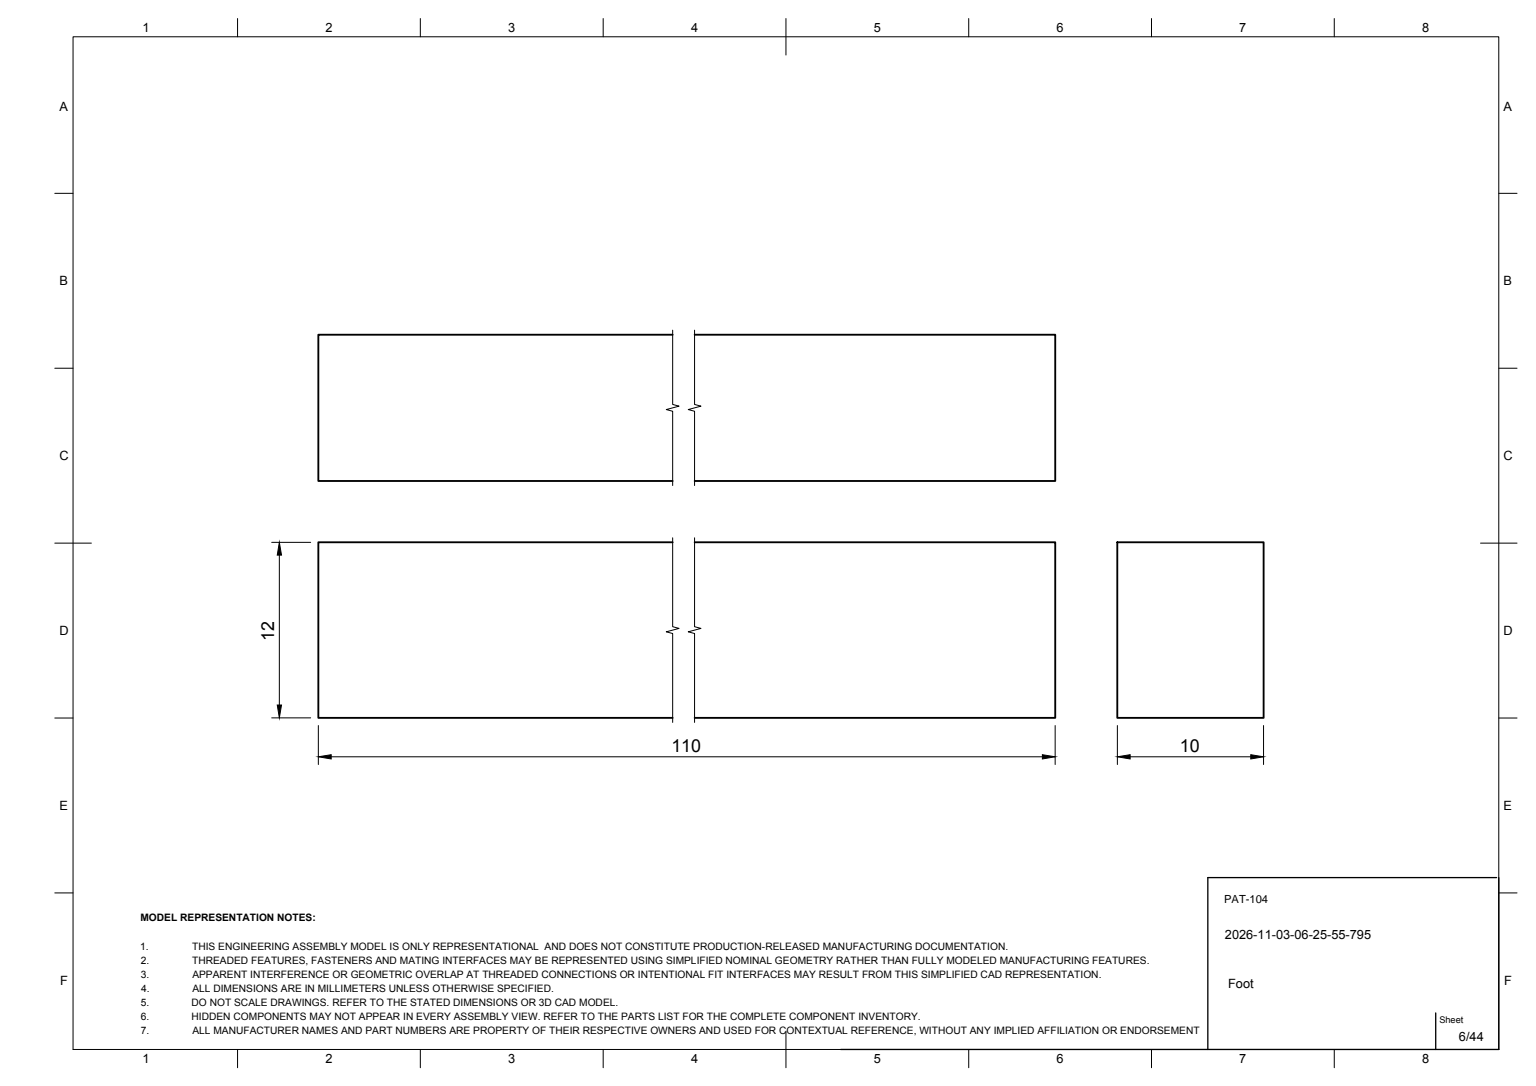
ISO-10303-21;
HEADER;
/* Generated by software containing ST-Developer
 * from STEP Tools, Inc. (www.steptools.com) 
 */

FILE_DESCRIPTION(
/* description */ ('Timing belt drive module 2 mm Pitch Timing 20T-40T'),

/* implementation_level */ '2;1');

FILE_NAME(
/* name */ 'Foot.step',
/* time_stamp */ '2026-10-28T03:25:12-07:00',
/* author */ (''),
/* organization */ (''),
/* preprocessor_version */ 'ST-DEVELOPER v20.2',
/* originating_system */ 'Autodesk Translation Framework v15.17.0.0',
/* authorisation */ '');

FILE_SCHEMA (('AUTOMOTIVE_DESIGN { 1 0 10303 214 3 1 1 }'));
ENDSEC;

DATA;
#10=MECHANICAL_DESIGN_GEOMETRIC_PRESENTATION_REPRESENTATION('',(#525),#17830);
#439=SHAPE_REPRESENTATION_RELATIONSHIP('SRR','None',#18009,#482);
#482=ADVANCED_BREP_SHAPE_REPRESENTATION('',(#583),#17784);
#525=STYLED_ITEM('',(#18331),#583);
#583=MANIFOLD_SOLID_BREP('Body1',#8982);
#791=PLANE('',#9578);
#792=PLANE('',#9579);
#793=PLANE('',#9580);
#794=PLANE('',#9581);
#795=PLANE('',#9582);
#796=PLANE('',#9583);
#992=FACE_OUTER_BOUND('',#1523,.T.);
#993=FACE_OUTER_BOUND('',#1524,.T.);
#994=FACE_OUTER_BOUND('',#1525,.T.);
#995=FACE_OUTER_BOUND('',#1526,.T.);
#996=FACE_OUTER_BOUND('',#1527,.T.);
#997=FACE_OUTER_BOUND('',#1528,.T.);
#1523=EDGE_LOOP('',(#5929,#5930,#5931,#5932));
#1524=EDGE_LOOP('',(#5933,#5934,#5935,#5936));
#1525=EDGE_LOOP('',(#5937,#5938,#5939,#5940));
#1526=EDGE_LOOP('',(#5941,#5942,#5943,#5944));
#1527=EDGE_LOOP('',(#5945,#5946,#5947,#5948));
#1528=EDGE_LOOP('',(#5949,#5950,#5951,#5952));
#2840=LINE('',#14040,#3318);
#2841=LINE('',#14042,#3319);
#2842=LINE('',#14044,#3320);
#2843=LINE('',#14045,#3321);
#2844=LINE('',#14048,#3322);
#2845=LINE('',#14050,#3323);
#2846=LINE('',#14051,#3324);
#2847=LINE('',#14054,#3325);
#2848=LINE('',#14056,#3326);
#2849=LINE('',#14057,#3327);
#2850=LINE('',#14059,#3328);
#2851=LINE('',#14060,#3329);
#3318=VECTOR('',#10985,1.);
#3319=VECTOR('',#10986,1.);
#3320=VECTOR('',#10987,1.);
#3321=VECTOR('',#10988,1.);
#3322=VECTOR('',#10991,1.);
#3323=VECTOR('',#10992,1.);
#3324=VECTOR('',#10993,1.);
#3325=VECTOR('',#10996,1.);
#3326=VECTOR('',#10997,1.);
#3327=VECTOR('',#10998,1.);
#3328=VECTOR('',#11001,1.);
#3329=VECTOR('',#11002,1.);
#3798=VERTEX_POINT('',#14038);
#3799=VERTEX_POINT('',#14039);
#3800=VERTEX_POINT('',#14041);
#3801=VERTEX_POINT('',#14043);
#3802=VERTEX_POINT('',#14047);
#3803=VERTEX_POINT('',#14049);
#3804=VERTEX_POINT('',#14053);
#3805=VERTEX_POINT('',#14055);
#4647=EDGE_CURVE('',#3798,#3799,#2840,.T.);
#4648=EDGE_CURVE('',#3799,#3800,#2841,.T.);
#4649=EDGE_CURVE('',#3801,#3800,#2842,.T.);
#4650=EDGE_CURVE('',#3798,#3801,#2843,.T.);
#4651=EDGE_CURVE('',#3802,#3798,#2844,.T.);
#4652=EDGE_CURVE('',#3803,#3801,#2845,.T.);
#4653=EDGE_CURVE('',#3802,#3803,#2846,.T.);
#4654=EDGE_CURVE('',#3804,#3802,#2847,.T.);
#4655=EDGE_CURVE('',#3805,#3803,#2848,.T.);
#4656=EDGE_CURVE('',#3804,#3805,#2849,.T.);
#4657=EDGE_CURVE('',#3799,#3804,#2850,.T.);
#4658=EDGE_CURVE('',#3800,#3805,#2851,.T.);
#5929=ORIENTED_EDGE('',*,*,#4647,.T.);
#5930=ORIENTED_EDGE('',*,*,#4648,.T.);
#5931=ORIENTED_EDGE('',*,*,#4649,.F.);
#5932=ORIENTED_EDGE('',*,*,#4650,.F.);
#5933=ORIENTED_EDGE('',*,*,#4651,.T.);
#5934=ORIENTED_EDGE('',*,*,#4650,.T.);
#5935=ORIENTED_EDGE('',*,*,#4652,.F.);
#5936=ORIENTED_EDGE('',*,*,#4653,.F.);
#5937=ORIENTED_EDGE('',*,*,#4654,.T.);
#5938=ORIENTED_EDGE('',*,*,#4653,.T.);
#5939=ORIENTED_EDGE('',*,*,#4655,.F.);
#5940=ORIENTED_EDGE('',*,*,#4656,.F.);
#5941=ORIENTED_EDGE('',*,*,#4657,.T.);
#5942=ORIENTED_EDGE('',*,*,#4656,.T.);
#5943=ORIENTED_EDGE('',*,*,#4658,.F.);
#5944=ORIENTED_EDGE('',*,*,#4648,.F.);
#5945=ORIENTED_EDGE('',*,*,#4658,.T.);
#5946=ORIENTED_EDGE('',*,*,#4655,.T.);
#5947=ORIENTED_EDGE('',*,*,#4652,.T.);
#5948=ORIENTED_EDGE('',*,*,#4649,.T.);
#5949=ORIENTED_EDGE('',*,*,#4657,.F.);
#5950=ORIENTED_EDGE('',*,*,#4647,.F.);
#5951=ORIENTED_EDGE('',*,*,#4651,.F.);
#5952=ORIENTED_EDGE('',*,*,#4654,.F.);
#8490=ADVANCED_FACE('',(#992),#791,.T.);
#8491=ADVANCED_FACE('',(#993),#792,.T.);
#8492=ADVANCED_FACE('',(#994),#793,.T.);
#8493=ADVANCED_FACE('',(#995),#794,.T.);
#8494=ADVANCED_FACE('',(#996),#795,.T.);
#8495=ADVANCED_FACE('',(#997),#796,.F.);
#8982=CLOSED_SHELL('',(#8490,#8491,#8492,#8493,#8494,#8495));
#9577=AXIS2_PLACEMENT_3D('',#14036,#10981,#10982);
#9578=AXIS2_PLACEMENT_3D('',#14037,#10983,#10984);
#9579=AXIS2_PLACEMENT_3D('',#14046,#10989,#10990);
#9580=AXIS2_PLACEMENT_3D('',#14052,#10994,#10995);
#9581=AXIS2_PLACEMENT_3D('',#14058,#10999,#11000);
#9582=AXIS2_PLACEMENT_3D('',#14061,#11003,#11004);
#9583=AXIS2_PLACEMENT_3D('',#14062,#11005,#11006);
#10981=DIRECTION('axis',(0.,0.,1.));
#10982=DIRECTION('refdir',(1.,0.,0.));
#10983=DIRECTION('center_axis',(0.,1.,0.));
#10984=DIRECTION('ref_axis',(-1.,0.,0.));
#10985=DIRECTION('',(-1.,0.,0.));
#10986=DIRECTION('',(0.,0.,1.));
#10987=DIRECTION('',(-1.,0.,0.));
#10988=DIRECTION('',(0.,0.,1.));
#10989=DIRECTION('center_axis',(1.,0.,0.));
#10990=DIRECTION('ref_axis',(0.,1.,0.));
#10991=DIRECTION('',(0.,1.,0.));
#10992=DIRECTION('',(0.,1.,0.));
#10993=DIRECTION('',(0.,0.,1.));
#10994=DIRECTION('center_axis',(0.,-1.,0.));
#10995=DIRECTION('ref_axis',(1.,0.,0.));
#10996=DIRECTION('',(1.,0.,0.));
#10997=DIRECTION('',(1.,0.,0.));
#10998=DIRECTION('',(0.,0.,1.));
#10999=DIRECTION('center_axis',(-1.,0.,0.));
#11000=DIRECTION('ref_axis',(0.,-1.,0.));
#11001=DIRECTION('',(0.,-1.,0.));
#11002=DIRECTION('',(0.,-1.,0.));
#11003=DIRECTION('center_axis',(0.,0.,1.));
#11004=DIRECTION('ref_axis',(1.,0.,0.));
#11005=DIRECTION('center_axis',(0.,0.,1.));
#11006=DIRECTION('ref_axis',(1.,0.,0.));
#14036=CARTESIAN_POINT('',(0.,0.,0.));
#14037=CARTESIAN_POINT('Origin',(-3.,4.5,-2.4));
#14038=CARTESIAN_POINT('',(-3.,4.5,-2.4));
#14039=CARTESIAN_POINT('',(-4.,4.5,-2.4));
#14040=CARTESIAN_POINT('',(-3.,4.5,-2.4));
#14041=CARTESIAN_POINT('',(-4.,4.5,-1.2));
#14042=CARTESIAN_POINT('',(-4.,4.5,-2.4));
#14043=CARTESIAN_POINT('',(-3.,4.5,-1.2));
#14044=CARTESIAN_POINT('',(-3.,4.5,-1.2));
#14045=CARTESIAN_POINT('',(-3.,4.5,-2.4));
#14046=CARTESIAN_POINT('Origin',(-3.,-6.5,-2.4));
#14047=CARTESIAN_POINT('',(-3.,-6.5,-2.4));
#14048=CARTESIAN_POINT('',(-3.,-6.5,-2.4));
#14049=CARTESIAN_POINT('',(-3.,-6.5,-1.2));
#14050=CARTESIAN_POINT('',(-3.,-6.5,-1.2));
#14051=CARTESIAN_POINT('',(-3.,-6.5,-2.4));
#14052=CARTESIAN_POINT('Origin',(-4.,-6.5,-2.4));
#14053=CARTESIAN_POINT('',(-4.,-6.5,-2.4));
#14054=CARTESIAN_POINT('',(-4.,-6.5,-2.4));
#14055=CARTESIAN_POINT('',(-4.,-6.5,-1.2));
#14056=CARTESIAN_POINT('',(-4.,-6.5,-1.2));
#14057=CARTESIAN_POINT('',(-4.,-6.5,-2.4));
#14058=CARTESIAN_POINT('Origin',(-4.,4.5,-2.4));
#14059=CARTESIAN_POINT('',(-4.,4.5,-2.4));
#14060=CARTESIAN_POINT('',(-4.,4.5,-1.2));
#14061=CARTESIAN_POINT('Origin',(-3.5,-1.,-1.2));
#14062=CARTESIAN_POINT('Origin',(-3.5,-1.,-2.4));
#17734=UNCERTAINTY_MEASURE_WITH_UNIT(LENGTH_MEASURE(0.001),#17831,
'DISTANCE_ACCURACY_VALUE',
'Maximum model space distance between geometric entities at asserted c
onnectivities');
#17780=UNCERTAINTY_MEASURE_WITH_UNIT(LENGTH_MEASURE(0.001),#17831,
'DISTANCE_ACCURACY_VALUE',
'Maximum model space distance between geometric entities at asserted c
onnectivities');
#17784=(
GEOMETRIC_REPRESENTATION_CONTEXT(3)
GLOBAL_UNCERTAINTY_ASSIGNED_CONTEXT((#17734))
GLOBAL_UNIT_ASSIGNED_CONTEXT((#17831,#17833,#17834))
REPRESENTATION_CONTEXT('','3D')
);
#17830=(
GEOMETRIC_REPRESENTATION_CONTEXT(3)
GLOBAL_UNCERTAINTY_ASSIGNED_CONTEXT((#17780))
GLOBAL_UNIT_ASSIGNED_CONTEXT((#17831,#17833,#17834))
REPRESENTATION_CONTEXT('','3D')
);
#17831=(
LENGTH_UNIT()
NAMED_UNIT(*)
SI_UNIT(.CENTI.,.METRE.)
);
#17833=(
NAMED_UNIT(*)
PLANE_ANGLE_UNIT()
SI_UNIT($,.RADIAN.)
);
#17834=(
NAMED_UNIT(*)
SI_UNIT($,.STERADIAN.)
SOLID_ANGLE_UNIT()
);
#17838=SHAPE_DEFINITION_REPRESENTATION(#17887,#18009);
#17887=PRODUCT_DEFINITION_SHAPE('',$,#18059);
#18009=SHAPE_REPRESENTATION('',(#9577),#17784);
#18055=PRODUCT_DEFINITION_CONTEXT('part definition',#18204,'design');
#18059=PRODUCT_DEFINITION('Foot','Foot',#18108,#18055);
#18108=PRODUCT_DEFINITION_FORMATION('',$,#18209);
#18204=APPLICATION_CONTEXT(
'Core Data for Automotive Mechanical Design Process');
#18205=PRODUCT_CONTEXT('part definition',#18204,'mechanical');
#18209=PRODUCT('Foot','Foot','Foot',(#18205));
#18325=COLOUR_RGB('Off White',0.89,0.88,0.83);
#18326=FILL_AREA_STYLE_COLOUR('',#18325);
#18327=FILL_AREA_STYLE('',(#18326));
#18328=SURFACE_STYLE_FILL_AREA(#18327);
#18329=SURFACE_SIDE_STYLE('',(#18328));
#18330=SURFACE_STYLE_USAGE(.BOTH.,#18329);
#18331=PRESENTATION_STYLE_ASSIGNMENT((#18330));
ENDSEC;
END-ISO-10303-21;
